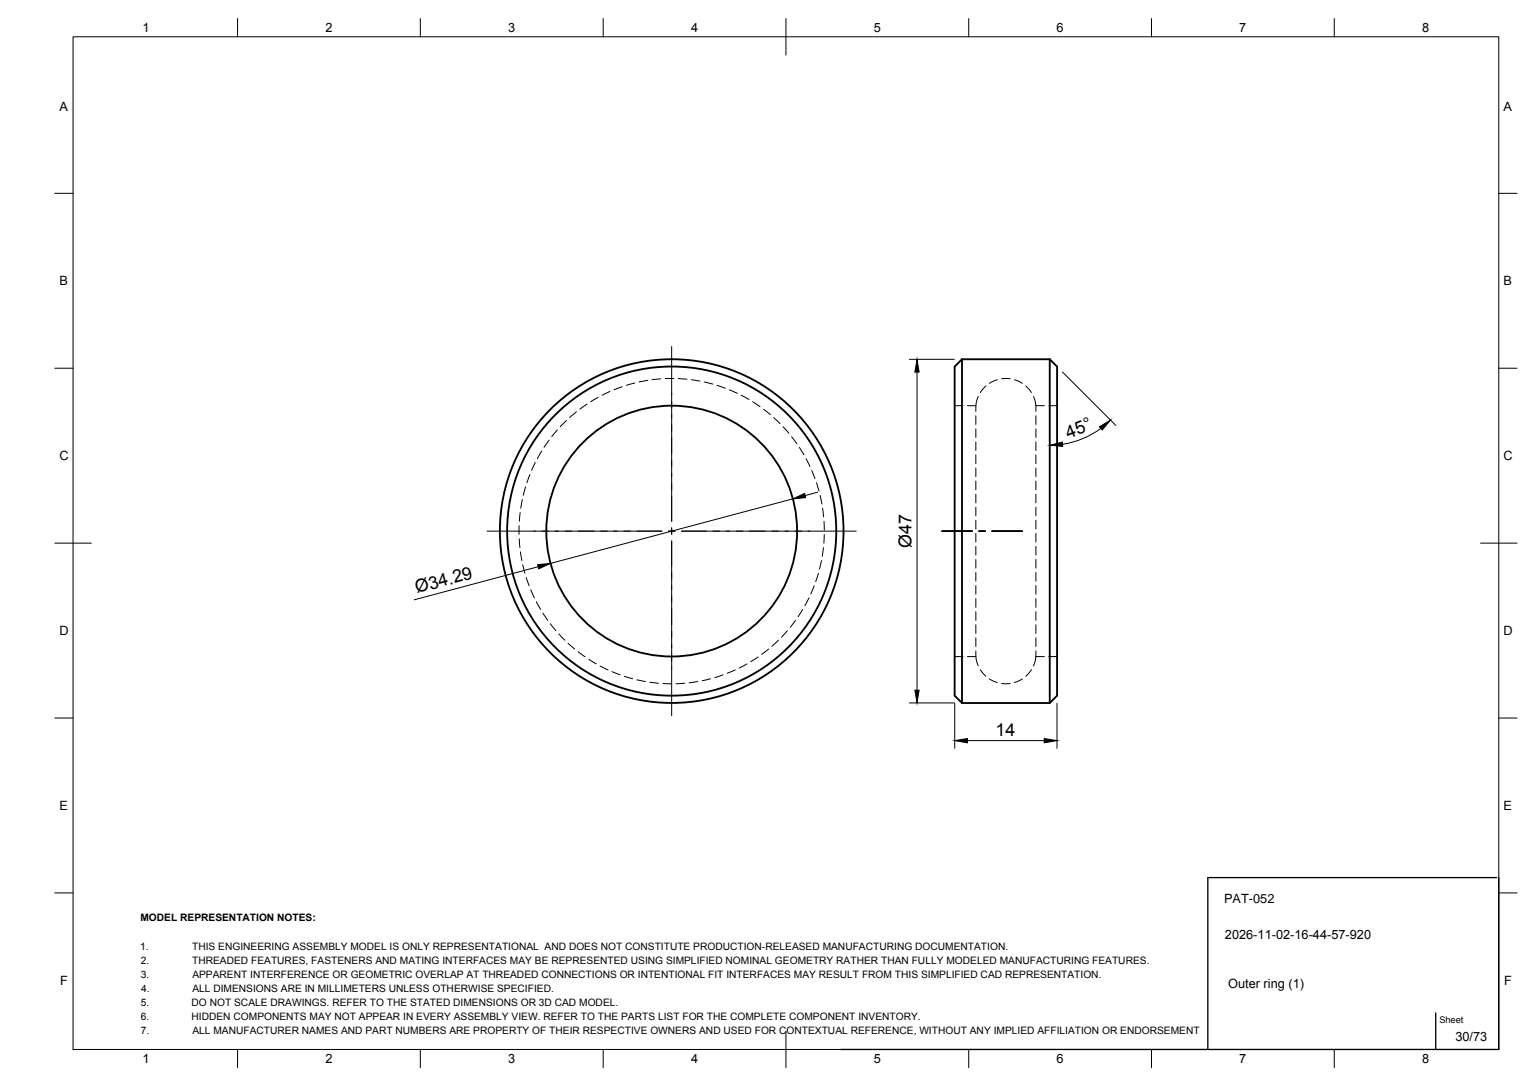
ISO-10303-21;
HEADER;
/* Generated by software containing ST-Developer
 * from STEP Tools, Inc. (www.steptools.com) 
 */

FILE_DESCRIPTION(
/* description */ ('Hand-crank gear train demonstrator'),
/* implementation_level */ '2;1');

FILE_NAME(
/* name */ 'Outer ring (1).step',
/* time_stamp */ '2026-10-28T03:22:13-07:00',
/* author */ (''),
/* organization */ (''),
/* preprocessor_version */ 'ST-DEVELOPER v20.2',
/* originating_system */ 'Autodesk Translation Framework v15.17.0.0',
/* authorisation */ '');

FILE_SCHEMA (('AUTOMOTIVE_DESIGN { 1 0 10303 214 3 1 1 }'));
ENDSEC;

DATA;
#10=MECHANICAL_DESIGN_GEOMETRIC_PRESENTATION_REPRESENTATION('',(#1213),#62758);
#1024=TOROIDAL_SURFACE('',#17634,1.675,0.412776);
#1034=CONICAL_SURFACE('',#17645,2.3,0.785398163397449);
#1035=CONICAL_SURFACE('',#17649,2.3,0.785398163397449);
#1078=SHAPE_REPRESENTATION_RELATIONSHIP('SRR','None',#63052,#1142);
#1142=ADVANCED_BREP_SHAPE_REPRESENTATION('',(#1291),#62706);
#1213=STYLED_ITEM('',(#63462),#1291);
#1291=MANIFOLD_SOLID_BREP('Body1',#16394);
#1498=FACE_BOUND('',#3412,.T.);
#1499=FACE_BOUND('',#3417,.T.);
#1700=PLANE('',#17642);
#1701=PLANE('',#17651);
#2317=FACE_OUTER_BOUND('',#3409,.T.);
#2318=FACE_OUTER_BOUND('',#3410,.T.);
#2319=FACE_OUTER_BOUND('',#3411,.T.);
#2320=FACE_OUTER_BOUND('',#3413,.T.);
#2321=FACE_OUTER_BOUND('',#3414,.T.);
#2322=FACE_OUTER_BOUND('',#3415,.T.);
#2323=FACE_OUTER_BOUND('',#3416,.T.);
#2324=FACE_OUTER_BOUND('',#3418,.T.);
#3409=EDGE_LOOP('',(#11689,#11690,#11691,#11692,#11693,#11694));
#3410=EDGE_LOOP('',(#11695,#11696,#11697,#11698,#11699));
#3411=EDGE_LOOP('',(#11700));
#3412=EDGE_LOOP('',(#11701));
#3413=EDGE_LOOP('',(#11702,#11703,#11704,#11705));
#3414=EDGE_LOOP('',(#11706,#11707,#11708,#11709));
#3415=EDGE_LOOP('',(#11710,#11711,#11712,#11713));
#3416=EDGE_LOOP('',(#11714));
#3417=EDGE_LOOP('',(#11715));
#3418=EDGE_LOOP('',(#11716,#11717,#11718,#11719,#11720));
#4444=LINE('',#24555,#5576);
#4445=LINE('',#24564,#5577);
#4446=LINE('',#24568,#5578);
#4447=LINE('',#24572,#5579);
#4448=LINE('',#24575,#5580);
#5576=VECTOR('',#19957,1.71469);
#5577=VECTOR('',#19968,2.3);
#5578=VECTOR('',#19973,2.35);
#5579=VECTOR('',#19978,2.3);
#5580=VECTOR('',#19983,1.71469);
#6805=CIRCLE('',#17635,1.71469);
#6806=CIRCLE('',#17636,1.71469);
#6807=CIRCLE('',#17637,0.412776);
#6808=CIRCLE('',#17638,1.71469);
#6809=CIRCLE('',#17639,1.71469);
#6810=CIRCLE('',#17641,1.71469);
#6811=CIRCLE('',#17643,2.25);
#6812=CIRCLE('',#17644,1.71469);
#6813=CIRCLE('',#17646,2.35);
#6814=CIRCLE('',#17648,2.35);
#6815=CIRCLE('',#17650,2.25);
#7503=VERTEX_POINT('',#24543);
#7504=VERTEX_POINT('',#24544);
#7505=VERTEX_POINT('',#24547);
#7506=VERTEX_POINT('',#24549);
#7507=VERTEX_POINT('',#24553);
#7508=VERTEX_POINT('',#24557);
#7509=VERTEX_POINT('',#24559);
#7510=VERTEX_POINT('',#24562);
#7511=VERTEX_POINT('',#24566);
#7512=VERTEX_POINT('',#24570);
#9096=EDGE_CURVE('',#7503,#7504,#6805,.T.);
#9097=EDGE_CURVE('',#7504,#7503,#6806,.T.);
#9098=EDGE_CURVE('',#7504,#7505,#6807,.T.);
#9099=EDGE_CURVE('',#7506,#7505,#6808,.T.);
#9100=EDGE_CURVE('',#7505,#7506,#6809,.T.);
#9101=EDGE_CURVE('',#7507,#7507,#6810,.T.);
#9102=EDGE_CURVE('',#7507,#7506,#4444,.T.);
#9103=EDGE_CURVE('',#7508,#7508,#6811,.T.);
#9104=EDGE_CURVE('',#7509,#7509,#6812,.T.);
#9105=EDGE_CURVE('',#7510,#7510,#6813,.T.);
#9106=EDGE_CURVE('',#7510,#7508,#4445,.T.);
#9107=EDGE_CURVE('',#7511,#7511,#6814,.T.);
#9108=EDGE_CURVE('',#7511,#7510,#4446,.T.);
#9109=EDGE_CURVE('',#7512,#7512,#6815,.T.);
#9110=EDGE_CURVE('',#7512,#7511,#4447,.T.);
#9111=EDGE_CURVE('',#7503,#7509,#4448,.T.);
#11689=ORIENTED_EDGE('',*,*,#9096,.F.);
#11690=ORIENTED_EDGE('',*,*,#9097,.F.);
#11691=ORIENTED_EDGE('',*,*,#9098,.T.);
#11692=ORIENTED_EDGE('',*,*,#9099,.F.);
#11693=ORIENTED_EDGE('',*,*,#9100,.F.);
#11694=ORIENTED_EDGE('',*,*,#9098,.F.);
#11695=ORIENTED_EDGE('',*,*,#9101,.T.);
#11696=ORIENTED_EDGE('',*,*,#9102,.T.);
#11697=ORIENTED_EDGE('',*,*,#9099,.T.);
#11698=ORIENTED_EDGE('',*,*,#9100,.T.);
#11699=ORIENTED_EDGE('',*,*,#9102,.F.);
#11700=ORIENTED_EDGE('',*,*,#9103,.F.);
#11701=ORIENTED_EDGE('',*,*,#9104,.T.);
#11702=ORIENTED_EDGE('',*,*,#9105,.F.);
#11703=ORIENTED_EDGE('',*,*,#9106,.T.);
#11704=ORIENTED_EDGE('',*,*,#9103,.T.);
#11705=ORIENTED_EDGE('',*,*,#9106,.F.);
#11706=ORIENTED_EDGE('',*,*,#9107,.F.);
#11707=ORIENTED_EDGE('',*,*,#9108,.T.);
#11708=ORIENTED_EDGE('',*,*,#9105,.T.);
#11709=ORIENTED_EDGE('',*,*,#9108,.F.);
#11710=ORIENTED_EDGE('',*,*,#9109,.F.);
#11711=ORIENTED_EDGE('',*,*,#9110,.T.);
#11712=ORIENTED_EDGE('',*,*,#9107,.T.);
#11713=ORIENTED_EDGE('',*,*,#9110,.F.);
#11714=ORIENTED_EDGE('',*,*,#9109,.T.);
#11715=ORIENTED_EDGE('',*,*,#9101,.F.);
#11716=ORIENTED_EDGE('',*,*,#9096,.T.);
#11717=ORIENTED_EDGE('',*,*,#9097,.T.);
#11718=ORIENTED_EDGE('',*,*,#9111,.T.);
#11719=ORIENTED_EDGE('',*,*,#9104,.F.);
#11720=ORIENTED_EDGE('',*,*,#9111,.F.);
#15268=CYLINDRICAL_SURFACE('',#17640,1.71469);
#15269=CYLINDRICAL_SURFACE('',#17647,2.35);
#15270=CYLINDRICAL_SURFACE('',#17652,1.71469);
#15627=ADVANCED_FACE('',(#2317),#1024,.F.);
#15628=ADVANCED_FACE('',(#2318),#15268,.F.);
#15629=ADVANCED_FACE('',(#2319,#1498),#1700,.T.);
#15630=ADVANCED_FACE('',(#2320),#1034,.T.);
#15631=ADVANCED_FACE('',(#2321),#15269,.T.);
#15632=ADVANCED_FACE('',(#2322),#1035,.T.);
#15633=ADVANCED_FACE('',(#2323,#1499),#1701,.T.);
#15634=ADVANCED_FACE('',(#2324),#15270,.F.);
#16394=CLOSED_SHELL('',(#15627,#15628,#15629,#15630,#15631,#15632,#15633,
#15634));
#17633=AXIS2_PLACEMENT_3D('',#24541,#19939,#19940);
#17634=AXIS2_PLACEMENT_3D('',#24542,#19941,#19942);
#17635=AXIS2_PLACEMENT_3D('',#24545,#19943,#19944);
#17636=AXIS2_PLACEMENT_3D('',#24546,#19945,#19946);
#17637=AXIS2_PLACEMENT_3D('',#24548,#19947,#19948);
#17638=AXIS2_PLACEMENT_3D('',#24550,#19949,#19950);
#17639=AXIS2_PLACEMENT_3D('',#24551,#19951,#19952);
#17640=AXIS2_PLACEMENT_3D('',#24552,#19953,#19954);
#17641=AXIS2_PLACEMENT_3D('',#24554,#19955,#19956);
#17642=AXIS2_PLACEMENT_3D('',#24556,#19958,#19959);
#17643=AXIS2_PLACEMENT_3D('',#24558,#19960,#19961);
#17644=AXIS2_PLACEMENT_3D('',#24560,#19962,#19963);
#17645=AXIS2_PLACEMENT_3D('',#24561,#19964,#19965);
#17646=AXIS2_PLACEMENT_3D('',#24563,#19966,#19967);
#17647=AXIS2_PLACEMENT_3D('',#24565,#19969,#19970);
#17648=AXIS2_PLACEMENT_3D('',#24567,#19971,#19972);
#17649=AXIS2_PLACEMENT_3D('',#24569,#19974,#19975);
#17650=AXIS2_PLACEMENT_3D('',#24571,#19976,#19977);
#17651=AXIS2_PLACEMENT_3D('',#24573,#19979,#19980);
#17652=AXIS2_PLACEMENT_3D('',#24574,#19981,#19982);
#19939=DIRECTION('axis',(0.,0.,1.));
#19940=DIRECTION('refdir',(1.,0.,0.));
#19941=DIRECTION('center_axis',(0.,-1.,0.));
#19942=DIRECTION('ref_axis',(0.,0.,-1.));
#19943=DIRECTION('center_axis',(0.,-1.,0.));
#19944=DIRECTION('ref_axis',(1.,0.,0.));
#19945=DIRECTION('center_axis',(0.,-1.,0.));
#19946=DIRECTION('ref_axis',(1.,0.,0.));
#19947=DIRECTION('center_axis',(1.,0.,1.22464679914735E-16));
#19948=DIRECTION('ref_axis',(-1.22464679914735E-16,0.,1.));
#19949=DIRECTION('center_axis',(0.,1.,0.));
#19950=DIRECTION('ref_axis',(1.,0.,0.));
#19951=DIRECTION('center_axis',(0.,1.,0.));
#19952=DIRECTION('ref_axis',(1.,0.,0.));
#19953=DIRECTION('center_axis',(0.,-1.,0.));
#19954=DIRECTION('ref_axis',(1.,0.,0.));
#19955=DIRECTION('center_axis',(0.,-1.,0.));
#19956=DIRECTION('ref_axis',(1.,0.,0.));
#19957=DIRECTION('',(0.,1.,0.));
#19958=DIRECTION('center_axis',(0.,1.,0.));
#19959=DIRECTION('ref_axis',(0.,0.,1.));
#19960=DIRECTION('center_axis',(0.,-1.,0.));
#19961=DIRECTION('ref_axis',(1.,0.,0.));
#19962=DIRECTION('center_axis',(0.,-1.,0.));
#19963=DIRECTION('ref_axis',(1.,0.,0.));
#19964=DIRECTION('center_axis',(0.,-1.,0.));
#19965=DIRECTION('ref_axis',(1.,0.,0.));
#19966=DIRECTION('center_axis',(0.,-1.,0.));
#19967=DIRECTION('ref_axis',(1.,0.,0.));
#19968=DIRECTION('',(0.707106781186548,0.707106781186547,8.65956056235494E-17));
#19969=DIRECTION('center_axis',(0.,-1.,0.));
#19970=DIRECTION('ref_axis',(1.,0.,0.));
#19971=DIRECTION('center_axis',(0.,-1.,0.));
#19972=DIRECTION('ref_axis',(1.,0.,0.));
#19973=DIRECTION('',(0.,1.,0.));
#19974=DIRECTION('center_axis',(0.,1.,0.));
#19975=DIRECTION('ref_axis',(1.,0.,0.));
#19976=DIRECTION('center_axis',(0.,-1.,0.));
#19977=DIRECTION('ref_axis',(1.,0.,0.));
#19978=DIRECTION('',(-0.707106781186548,0.707106781186547,-8.65956056235494E-17));
#19979=DIRECTION('center_axis',(0.,-1.,0.));
#19980=DIRECTION('ref_axis',(0.,0.,-1.));
#19981=DIRECTION('center_axis',(0.,-1.,0.));
#19982=DIRECTION('ref_axis',(1.,0.,0.));
#19983=DIRECTION('',(0.,1.,0.));
#24541=CARTESIAN_POINT('',(0.,0.,0.));
#24542=CARTESIAN_POINT('Origin',(0.,0.,0.));
#24543=CARTESIAN_POINT('',(-1.71469,0.410863395882378,-2.09988962002998E-16));
#24544=CARTESIAN_POINT('',(-2.09988962002998E-16,0.410863395882378,1.71469));
#24545=CARTESIAN_POINT('Origin',(0.,0.410863395882378,0.));
#24546=CARTESIAN_POINT('Origin',(0.,0.410863395882378,0.));
#24547=CARTESIAN_POINT('',(-2.09988962002998E-16,-0.410863395882378,1.71469));
#24548=CARTESIAN_POINT('Origin',(-2.05128338857182E-16,0.,1.675));
#24549=CARTESIAN_POINT('',(-1.71469,-0.410863395882378,2.09988962002998E-16));
#24550=CARTESIAN_POINT('Origin',(0.,-0.410863395882378,0.));
#24551=CARTESIAN_POINT('Origin',(0.,-0.410863395882378,0.));
#24552=CARTESIAN_POINT('Origin',(0.,0.,0.));
#24553=CARTESIAN_POINT('',(-1.71469,-0.7,-2.09988962002998E-16));
#24554=CARTESIAN_POINT('Origin',(0.,-0.7,0.));
#24555=CARTESIAN_POINT('',(-1.71469,0.,-2.09988962002998E-16));
#24556=CARTESIAN_POINT('Origin',(2.25,0.7,0.));
#24557=CARTESIAN_POINT('',(-2.25,0.7,-2.75545529808154E-16));
#24558=CARTESIAN_POINT('Origin',(0.,0.7,0.));
#24559=CARTESIAN_POINT('',(-1.71469,0.7,-2.09988962002998E-16));
#24560=CARTESIAN_POINT('Origin',(0.,0.7,0.));
#24561=CARTESIAN_POINT('Origin',(0.,0.65,0.));
#24562=CARTESIAN_POINT('',(-2.35,0.6,-2.87791997799628E-16));
#24563=CARTESIAN_POINT('Origin',(0.,0.6,0.));
#24564=CARTESIAN_POINT('',(-2.3,0.65,-2.81668763803891E-16));
#24565=CARTESIAN_POINT('Origin',(0.,0.,0.));
#24566=CARTESIAN_POINT('',(-2.35,-0.6,-2.87791997799628E-16));
#24567=CARTESIAN_POINT('Origin',(0.,-0.6,0.));
#24568=CARTESIAN_POINT('',(-2.35,0.,-2.87791997799628E-16));
#24569=CARTESIAN_POINT('Origin',(0.,-0.65,0.));
#24570=CARTESIAN_POINT('',(-2.25,-0.7,-2.75545529808154E-16));
#24571=CARTESIAN_POINT('Origin',(0.,-0.7,0.));
#24572=CARTESIAN_POINT('',(-2.3,-0.65,-2.81668763803891E-16));
#24573=CARTESIAN_POINT('Origin',(1.71469,-0.7,0.));
#24574=CARTESIAN_POINT('Origin',(0.,0.,0.));
#24575=CARTESIAN_POINT('',(-1.71469,0.,-2.09988962002998E-16));
#62632=UNCERTAINTY_MEASURE_WITH_UNIT(LENGTH_MEASURE(0.001),#62759,
'DISTANCE_ACCURACY_VALUE',
'Maximum model space distance between geometric entities at asserted c
onnectivities');
#62684=UNCERTAINTY_MEASURE_WITH_UNIT(LENGTH_MEASURE(0.001),#62759,
'DISTANCE_ACCURACY_VALUE',
'Maximum model space distance between geometric entities at asserted c
onnectivities');
#62706=(
GEOMETRIC_REPRESENTATION_CONTEXT(3)
GLOBAL_UNCERTAINTY_ASSIGNED_CONTEXT((#62632))
GLOBAL_UNIT_ASSIGNED_CONTEXT((#62759,#62761,#62762))
REPRESENTATION_CONTEXT('','3D')
);
#62758=(
GEOMETRIC_REPRESENTATION_CONTEXT(3)
GLOBAL_UNCERTAINTY_ASSIGNED_CONTEXT((#62684))
GLOBAL_UNIT_ASSIGNED_CONTEXT((#62759,#62761,#62762))
REPRESENTATION_CONTEXT('','3D')
);
#62759=(
LENGTH_UNIT()
NAMED_UNIT(*)
SI_UNIT(.CENTI.,.METRE.)
);
#62761=(
NAMED_UNIT(*)
PLANE_ANGLE_UNIT()
SI_UNIT($,.RADIAN.)
);
#62762=(
NAMED_UNIT(*)
SI_UNIT($,.STERADIAN.)
SOLID_ANGLE_UNIT()
);
#62784=SHAPE_DEFINITION_REPRESENTATION(#62862,#63052);
#62862=PRODUCT_DEFINITION_SHAPE('',$,#63126);
#63052=SHAPE_REPRESENTATION('',(#17633),#62706);
#63104=PRODUCT_DEFINITION_CONTEXT('part definition',#63325,'design');
#63126=PRODUCT_DEFINITION('Outer ring (1)','Outer ring (1)',#63199,#63104);
#63199=PRODUCT_DEFINITION_FORMATION('',$,#63348);
#63325=APPLICATION_CONTEXT(
'Core Data for Automotive Mechanical Design Process');
#63326=PRODUCT_CONTEXT('part definition',#63325,'mechanical');
#63348=PRODUCT('Outer ring (1)','Outer ring (1)','Outer ring (1)',(#63326));
#63456=COLOUR_RGB('Grey',0.48,0.52,0.57);
#63457=FILL_AREA_STYLE_COLOUR('',#63456);
#63458=FILL_AREA_STYLE('',(#63457));
#63459=SURFACE_STYLE_FILL_AREA(#63458);
#63460=SURFACE_SIDE_STYLE('',(#63459));
#63461=SURFACE_STYLE_USAGE(.BOTH.,#63460);
#63462=PRESENTATION_STYLE_ASSIGNMENT((#63461));
ENDSEC;
END-ISO-10303-21;
